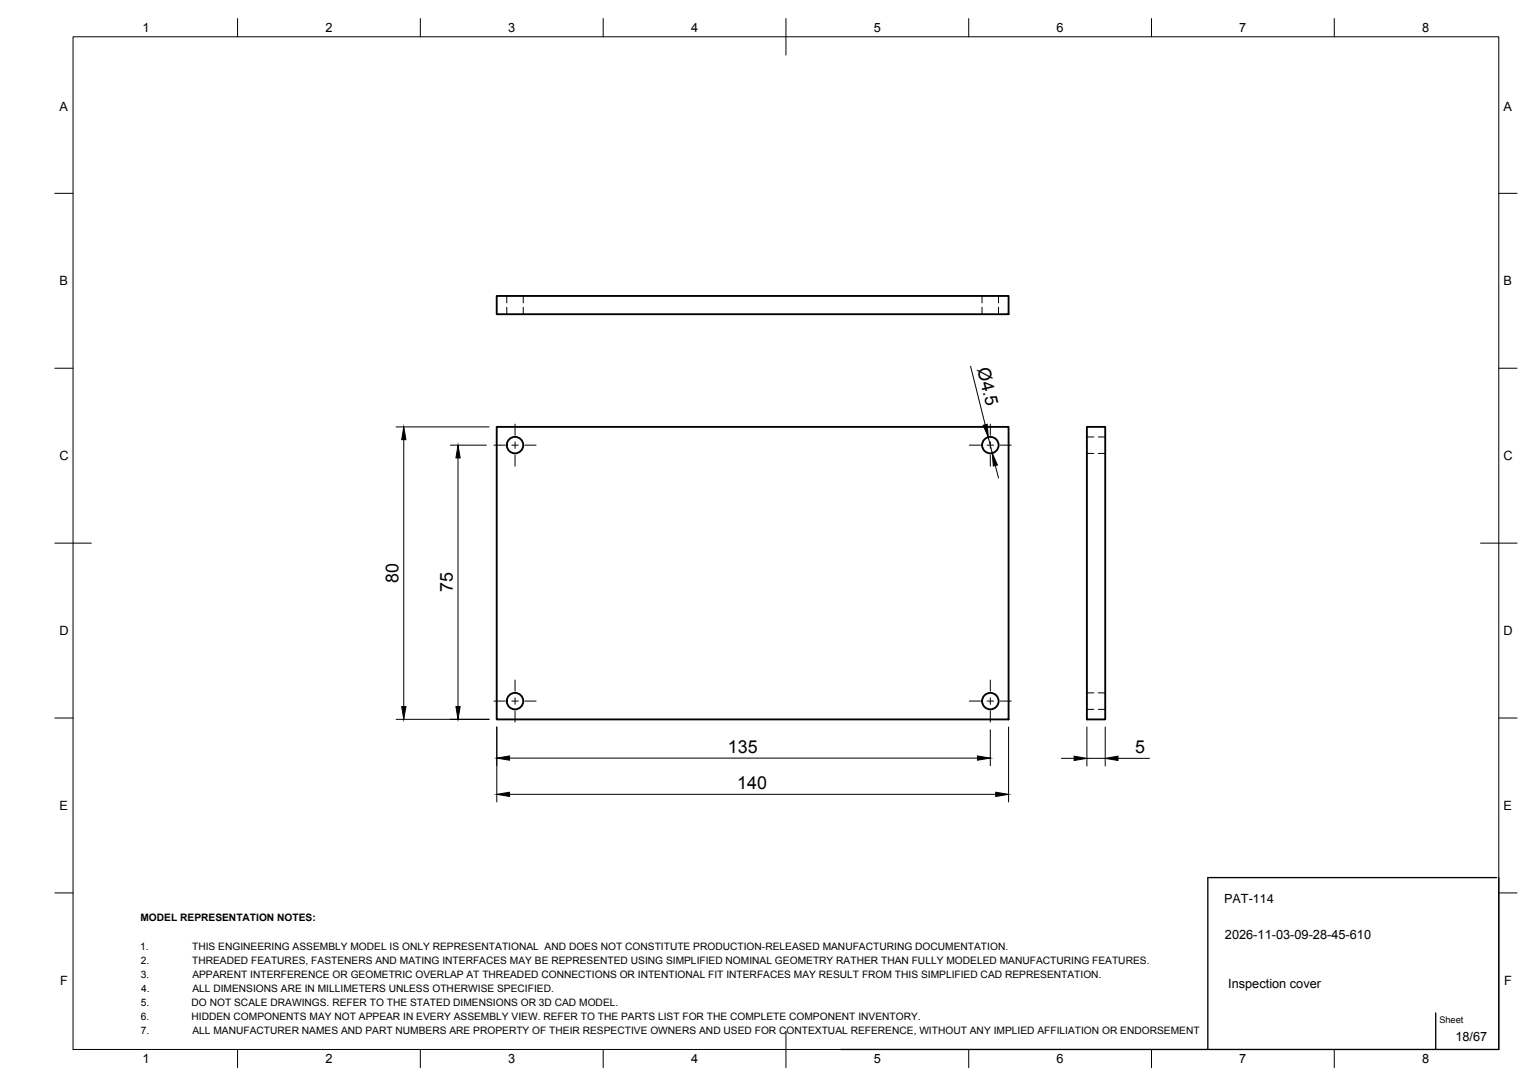
ISO-10303-21;
HEADER;
/* Generated by software containing ST-Developer
 * from STEP Tools, Inc. (www.steptools.com) 
 */

FILE_DESCRIPTION(
/* description */ ('Two-stage gear reducer in split housing'),
/* implementation_level */ '2;1');

FILE_NAME(
/* name */ 'Inspection cover.step',
/* time_stamp */ '2026-10-28T03:22:31-07:00',
/* author */ (''),
/* organization */ (''),
/* preprocessor_version */ 'ST-DEVELOPER v20.2',
/* originating_system */ 'Autodesk Translation Framework v15.17.0.0',
/* authorisation */ '');

FILE_SCHEMA (('AUTOMOTIVE_DESIGN { 1 0 10303 214 3 1 1 }'));
ENDSEC;

DATA;
#10=MECHANICAL_DESIGN_GEOMETRIC_PRESENTATION_REPRESENTATION('',(#1247),#73366);
#1135=SHAPE_REPRESENTATION_RELATIONSHIP('SRR','None',#73622,#1191);
#1191=ADVANCED_BREP_SHAPE_REPRESENTATION('',(#1318),#73318);
#1247=STYLED_ITEM('',(#73974),#1318);
#1318=MANIFOLD_SOLID_BREP('Body1',#16135);
#1510=FACE_BOUND('',#3320,.T.);
#1511=FACE_BOUND('',#3321,.T.);
#1512=FACE_BOUND('',#3322,.T.);
#1513=FACE_BOUND('',#3323,.T.);
#1514=FACE_BOUND('',#3325,.T.);
#1515=FACE_BOUND('',#3326,.T.);
#1516=FACE_BOUND('',#3327,.T.);
#1517=FACE_BOUND('',#3328,.T.);
#1726=PLANE('',#17372);
#1727=PLANE('',#17373);
#1728=PLANE('',#17374);
#1729=PLANE('',#17375);
#1730=PLANE('',#17376);
#1731=PLANE('',#17377);
#2262=FACE_OUTER_BOUND('',#3311,.T.);
#2263=FACE_OUTER_BOUND('',#3312,.T.);
#2264=FACE_OUTER_BOUND('',#3313,.T.);
#2265=FACE_OUTER_BOUND('',#3314,.T.);
#2266=FACE_OUTER_BOUND('',#3315,.T.);
#2267=FACE_OUTER_BOUND('',#3316,.T.);
#2268=FACE_OUTER_BOUND('',#3317,.T.);
#2269=FACE_OUTER_BOUND('',#3318,.T.);
#2270=FACE_OUTER_BOUND('',#3319,.T.);
#2271=FACE_OUTER_BOUND('',#3324,.T.);
#3311=EDGE_LOOP('',(#11659,#11660,#11661,#11662));
#3312=EDGE_LOOP('',(#11663,#11664,#11665,#11666));
#3313=EDGE_LOOP('',(#11667,#11668,#11669,#11670));
#3314=EDGE_LOOP('',(#11671,#11672,#11673,#11674));
#3315=EDGE_LOOP('',(#11675,#11676,#11677,#11678));
#3316=EDGE_LOOP('',(#11679,#11680,#11681,#11682));
#3317=EDGE_LOOP('',(#11683,#11684,#11685,#11686));
#3318=EDGE_LOOP('',(#11687,#11688,#11689,#11690));
#3319=EDGE_LOOP('',(#11691,#11692,#11693,#11694));
#3320=EDGE_LOOP('',(#11695));
#3321=EDGE_LOOP('',(#11696));
#3322=EDGE_LOOP('',(#11697));
#3323=EDGE_LOOP('',(#11698));
#3324=EDGE_LOOP('',(#11699,#11700,#11701,#11702));
#3325=EDGE_LOOP('',(#11703));
#3326=EDGE_LOOP('',(#11704));
#3327=EDGE_LOOP('',(#11705));
#3328=EDGE_LOOP('',(#11706));
#4360=LINE('',#24014,#5384);
#4361=LINE('',#24020,#5385);
#4362=LINE('',#24026,#5386);
#4363=LINE('',#24032,#5387);
#4364=LINE('',#24037,#5388);
#4365=LINE('',#24039,#5389);
#4366=LINE('',#24041,#5390);
#4367=LINE('',#24042,#5391);
#4368=LINE('',#24045,#5392);
#4369=LINE('',#24047,#5393);
#4370=LINE('',#24048,#5394);
#4371=LINE('',#24051,#5395);
#4372=LINE('',#24053,#5396);
#4373=LINE('',#24054,#5397);
#4374=LINE('',#24056,#5398);
#4375=LINE('',#24057,#5399);
#5384=VECTOR('',#19862,0.225);
#5385=VECTOR('',#19869,0.225);
#5386=VECTOR('',#19876,0.225);
#5387=VECTOR('',#19883,0.225);
#5388=VECTOR('',#19888,1.);
#5389=VECTOR('',#19889,1.);
#5390=VECTOR('',#19890,1.);
#5391=VECTOR('',#19891,1.);
#5392=VECTOR('',#19894,1.);
#5393=VECTOR('',#19895,1.);
#5394=VECTOR('',#19896,1.);
#5395=VECTOR('',#19899,1.);
#5396=VECTOR('',#19900,1.);
#5397=VECTOR('',#19901,1.);
#5398=VECTOR('',#19904,1.);
#5399=VECTOR('',#19905,1.);
#6376=CIRCLE('',#17361,0.225);
#6377=CIRCLE('',#17362,0.225);
#6378=CIRCLE('',#17364,0.225);
#6379=CIRCLE('',#17365,0.225);
#6380=CIRCLE('',#17367,0.225);
#6381=CIRCLE('',#17368,0.225);
#6382=CIRCLE('',#17370,0.225);
#6383=CIRCLE('',#17371,0.225);
#7208=VERTEX_POINT('',#24011);
#7209=VERTEX_POINT('',#24013);
#7210=VERTEX_POINT('',#24017);
#7211=VERTEX_POINT('',#24019);
#7212=VERTEX_POINT('',#24023);
#7213=VERTEX_POINT('',#24025);
#7214=VERTEX_POINT('',#24029);
#7215=VERTEX_POINT('',#24031);
#7216=VERTEX_POINT('',#24035);
#7217=VERTEX_POINT('',#24036);
#7218=VERTEX_POINT('',#24038);
#7219=VERTEX_POINT('',#24040);
#7220=VERTEX_POINT('',#24044);
#7221=VERTEX_POINT('',#24046);
#7222=VERTEX_POINT('',#24050);
#7223=VERTEX_POINT('',#24052);
#8883=EDGE_CURVE('',#7208,#7208,#6376,.T.);
#8884=EDGE_CURVE('',#7208,#7209,#4360,.T.);
#8885=EDGE_CURVE('',#7209,#7209,#6377,.T.);
#8886=EDGE_CURVE('',#7210,#7210,#6378,.T.);
#8887=EDGE_CURVE('',#7210,#7211,#4361,.T.);
#8888=EDGE_CURVE('',#7211,#7211,#6379,.T.);
#8889=EDGE_CURVE('',#7212,#7212,#6380,.T.);
#8890=EDGE_CURVE('',#7212,#7213,#4362,.T.);
#8891=EDGE_CURVE('',#7213,#7213,#6381,.T.);
#8892=EDGE_CURVE('',#7214,#7214,#6382,.T.);
#8893=EDGE_CURVE('',#7214,#7215,#4363,.T.);
#8894=EDGE_CURVE('',#7215,#7215,#6383,.T.);
#8895=EDGE_CURVE('',#7216,#7217,#4364,.T.);
#8896=EDGE_CURVE('',#7217,#7218,#4365,.T.);
#8897=EDGE_CURVE('',#7219,#7218,#4366,.T.);
#8898=EDGE_CURVE('',#7216,#7219,#4367,.T.);
#8899=EDGE_CURVE('',#7220,#7216,#4368,.T.);
#8900=EDGE_CURVE('',#7221,#7219,#4369,.T.);
#8901=EDGE_CURVE('',#7220,#7221,#4370,.T.);
#8902=EDGE_CURVE('',#7222,#7220,#4371,.T.);
#8903=EDGE_CURVE('',#7223,#7221,#4372,.T.);
#8904=EDGE_CURVE('',#7222,#7223,#4373,.T.);
#8905=EDGE_CURVE('',#7217,#7222,#4374,.T.);
#8906=EDGE_CURVE('',#7218,#7223,#4375,.T.);
#11659=ORIENTED_EDGE('',*,*,#8883,.F.);
#11660=ORIENTED_EDGE('',*,*,#8884,.T.);
#11661=ORIENTED_EDGE('',*,*,#8885,.F.);
#11662=ORIENTED_EDGE('',*,*,#8884,.F.);
#11663=ORIENTED_EDGE('',*,*,#8886,.F.);
#11664=ORIENTED_EDGE('',*,*,#8887,.T.);
#11665=ORIENTED_EDGE('',*,*,#8888,.F.);
#11666=ORIENTED_EDGE('',*,*,#8887,.F.);
#11667=ORIENTED_EDGE('',*,*,#8889,.F.);
#11668=ORIENTED_EDGE('',*,*,#8890,.T.);
#11669=ORIENTED_EDGE('',*,*,#8891,.F.);
#11670=ORIENTED_EDGE('',*,*,#8890,.F.);
#11671=ORIENTED_EDGE('',*,*,#8892,.F.);
#11672=ORIENTED_EDGE('',*,*,#8893,.T.);
#11673=ORIENTED_EDGE('',*,*,#8894,.F.);
#11674=ORIENTED_EDGE('',*,*,#8893,.F.);
#11675=ORIENTED_EDGE('',*,*,#8895,.T.);
#11676=ORIENTED_EDGE('',*,*,#8896,.T.);
#11677=ORIENTED_EDGE('',*,*,#8897,.F.);
#11678=ORIENTED_EDGE('',*,*,#8898,.F.);
#11679=ORIENTED_EDGE('',*,*,#8899,.T.);
#11680=ORIENTED_EDGE('',*,*,#8898,.T.);
#11681=ORIENTED_EDGE('',*,*,#8900,.F.);
#11682=ORIENTED_EDGE('',*,*,#8901,.F.);
#11683=ORIENTED_EDGE('',*,*,#8902,.T.);
#11684=ORIENTED_EDGE('',*,*,#8901,.T.);
#11685=ORIENTED_EDGE('',*,*,#8903,.F.);
#11686=ORIENTED_EDGE('',*,*,#8904,.F.);
#11687=ORIENTED_EDGE('',*,*,#8905,.T.);
#11688=ORIENTED_EDGE('',*,*,#8904,.T.);
#11689=ORIENTED_EDGE('',*,*,#8906,.F.);
#11690=ORIENTED_EDGE('',*,*,#8896,.F.);
#11691=ORIENTED_EDGE('',*,*,#8906,.T.);
#11692=ORIENTED_EDGE('',*,*,#8903,.T.);
#11693=ORIENTED_EDGE('',*,*,#8900,.T.);
#11694=ORIENTED_EDGE('',*,*,#8897,.T.);
#11695=ORIENTED_EDGE('',*,*,#8885,.T.);
#11696=ORIENTED_EDGE('',*,*,#8888,.T.);
#11697=ORIENTED_EDGE('',*,*,#8891,.T.);
#11698=ORIENTED_EDGE('',*,*,#8894,.T.);
#11699=ORIENTED_EDGE('',*,*,#8905,.F.);
#11700=ORIENTED_EDGE('',*,*,#8895,.F.);
#11701=ORIENTED_EDGE('',*,*,#8899,.F.);
#11702=ORIENTED_EDGE('',*,*,#8902,.F.);
#11703=ORIENTED_EDGE('',*,*,#8883,.T.);
#11704=ORIENTED_EDGE('',*,*,#8886,.T.);
#11705=ORIENTED_EDGE('',*,*,#8889,.T.);
#11706=ORIENTED_EDGE('',*,*,#8892,.T.);
#15043=CYLINDRICAL_SURFACE('',#17360,0.225);
#15044=CYLINDRICAL_SURFACE('',#17363,0.225);
#15045=CYLINDRICAL_SURFACE('',#17366,0.225);
#15046=CYLINDRICAL_SURFACE('',#17369,0.225);
#15469=ADVANCED_FACE('',(#2262),#15043,.F.);
#15470=ADVANCED_FACE('',(#2263),#15044,.F.);
#15471=ADVANCED_FACE('',(#2264),#15045,.F.);
#15472=ADVANCED_FACE('',(#2265),#15046,.F.);
#15473=ADVANCED_FACE('',(#2266),#1726,.T.);
#15474=ADVANCED_FACE('',(#2267),#1727,.T.);
#15475=ADVANCED_FACE('',(#2268),#1728,.T.);
#15476=ADVANCED_FACE('',(#2269),#1729,.T.);
#15477=ADVANCED_FACE('',(#2270,#1510,#1511,#1512,#1513),#1730,.T.);
#15478=ADVANCED_FACE('',(#2271,#1514,#1515,#1516,#1517),#1731,.F.);
#16135=CLOSED_SHELL('',(#15469,#15470,#15471,#15472,#15473,#15474,#15475,
#15476,#15477,#15478));
#17359=AXIS2_PLACEMENT_3D('',#24009,#19856,#19857);
#17360=AXIS2_PLACEMENT_3D('',#24010,#19858,#19859);
#17361=AXIS2_PLACEMENT_3D('',#24012,#19860,#19861);
#17362=AXIS2_PLACEMENT_3D('',#24015,#19863,#19864);
#17363=AXIS2_PLACEMENT_3D('',#24016,#19865,#19866);
#17364=AXIS2_PLACEMENT_3D('',#24018,#19867,#19868);
#17365=AXIS2_PLACEMENT_3D('',#24021,#19870,#19871);
#17366=AXIS2_PLACEMENT_3D('',#24022,#19872,#19873);
#17367=AXIS2_PLACEMENT_3D('',#24024,#19874,#19875);
#17368=AXIS2_PLACEMENT_3D('',#24027,#19877,#19878);
#17369=AXIS2_PLACEMENT_3D('',#24028,#19879,#19880);
#17370=AXIS2_PLACEMENT_3D('',#24030,#19881,#19882);
#17371=AXIS2_PLACEMENT_3D('',#24033,#19884,#19885);
#17372=AXIS2_PLACEMENT_3D('',#24034,#19886,#19887);
#17373=AXIS2_PLACEMENT_3D('',#24043,#19892,#19893);
#17374=AXIS2_PLACEMENT_3D('',#24049,#19897,#19898);
#17375=AXIS2_PLACEMENT_3D('',#24055,#19902,#19903);
#17376=AXIS2_PLACEMENT_3D('',#24058,#19906,#19907);
#17377=AXIS2_PLACEMENT_3D('',#24059,#19908,#19909);
#19856=DIRECTION('axis',(0.,0.,1.));
#19857=DIRECTION('refdir',(1.,0.,0.));
#19858=DIRECTION('center_axis',(0.,0.,1.));
#19859=DIRECTION('ref_axis',(1.,0.,0.));
#19860=DIRECTION('center_axis',(0.,0.,1.));
#19861=DIRECTION('ref_axis',(1.,0.,0.));
#19862=DIRECTION('',(0.,0.,1.));
#19863=DIRECTION('center_axis',(0.,0.,-1.));
#19864=DIRECTION('ref_axis',(1.,0.,0.));
#19865=DIRECTION('center_axis',(0.,0.,1.));
#19866=DIRECTION('ref_axis',(1.,0.,0.));
#19867=DIRECTION('center_axis',(0.,0.,1.));
#19868=DIRECTION('ref_axis',(1.,0.,0.));
#19869=DIRECTION('',(0.,0.,1.));
#19870=DIRECTION('center_axis',(0.,0.,-1.));
#19871=DIRECTION('ref_axis',(1.,0.,0.));
#19872=DIRECTION('center_axis',(0.,0.,1.));
#19873=DIRECTION('ref_axis',(1.,0.,0.));
#19874=DIRECTION('center_axis',(0.,0.,1.));
#19875=DIRECTION('ref_axis',(1.,0.,0.));
#19876=DIRECTION('',(0.,0.,1.));
#19877=DIRECTION('center_axis',(0.,0.,-1.));
#19878=DIRECTION('ref_axis',(1.,0.,0.));
#19879=DIRECTION('center_axis',(0.,0.,1.));
#19880=DIRECTION('ref_axis',(1.,0.,0.));
#19881=DIRECTION('center_axis',(0.,0.,1.));
#19882=DIRECTION('ref_axis',(1.,0.,0.));
#19883=DIRECTION('',(0.,0.,1.));
#19884=DIRECTION('center_axis',(0.,0.,-1.));
#19885=DIRECTION('ref_axis',(1.,0.,0.));
#19886=DIRECTION('center_axis',(0.,1.,0.));
#19887=DIRECTION('ref_axis',(-1.,0.,0.));
#19888=DIRECTION('',(-1.,0.,0.));
#19889=DIRECTION('',(0.,0.,1.));
#19890=DIRECTION('',(-1.,0.,0.));
#19891=DIRECTION('',(0.,0.,1.));
#19892=DIRECTION('center_axis',(1.,0.,0.));
#19893=DIRECTION('ref_axis',(0.,1.,0.));
#19894=DIRECTION('',(0.,1.,0.));
#19895=DIRECTION('',(0.,1.,0.));
#19896=DIRECTION('',(0.,0.,1.));
#19897=DIRECTION('center_axis',(0.,-1.,0.));
#19898=DIRECTION('ref_axis',(1.,0.,0.));
#19899=DIRECTION('',(1.,0.,0.));
#19900=DIRECTION('',(1.,0.,0.));
#19901=DIRECTION('',(0.,0.,1.));
#19902=DIRECTION('center_axis',(-1.,0.,0.));
#19903=DIRECTION('ref_axis',(0.,-1.,0.));
#19904=DIRECTION('',(0.,-1.,0.));
#19905=DIRECTION('',(0.,-1.,0.));
#19906=DIRECTION('center_axis',(0.,0.,1.));
#19907=DIRECTION('ref_axis',(1.,0.,0.));
#19908=DIRECTION('center_axis',(0.,0.,1.));
#19909=DIRECTION('ref_axis',(1.,0.,0.));
#24009=CARTESIAN_POINT('',(0.,0.,0.));
#24010=CARTESIAN_POINT('Origin',(14.5,-3.5,15.9));
#24011=CARTESIAN_POINT('',(14.275,-3.5,16.));
#24012=CARTESIAN_POINT('Origin',(14.5,-3.5,16.));
#24013=CARTESIAN_POINT('',(14.275,-3.5,16.5));
#24014=CARTESIAN_POINT('',(14.275,-3.5,15.9));
#24015=CARTESIAN_POINT('Origin',(14.5,-3.5,16.5));
#24016=CARTESIAN_POINT('Origin',(1.5,3.5,15.9));
#24017=CARTESIAN_POINT('',(1.275,3.5,16.));
#24018=CARTESIAN_POINT('Origin',(1.5,3.5,16.));
#24019=CARTESIAN_POINT('',(1.275,3.5,16.5));
#24020=CARTESIAN_POINT('',(1.275,3.5,15.9));
#24021=CARTESIAN_POINT('Origin',(1.5,3.5,16.5));
#24022=CARTESIAN_POINT('Origin',(1.5,-3.5,15.9));
#24023=CARTESIAN_POINT('',(1.275,-3.5,16.));
#24024=CARTESIAN_POINT('Origin',(1.5,-3.5,16.));
#24025=CARTESIAN_POINT('',(1.275,-3.5,16.5));
#24026=CARTESIAN_POINT('',(1.275,-3.5,15.9));
#24027=CARTESIAN_POINT('Origin',(1.5,-3.5,16.5));
#24028=CARTESIAN_POINT('Origin',(14.5,3.5,15.9));
#24029=CARTESIAN_POINT('',(14.275,3.5,16.));
#24030=CARTESIAN_POINT('Origin',(14.5,3.5,16.));
#24031=CARTESIAN_POINT('',(14.275,3.5,16.5));
#24032=CARTESIAN_POINT('',(14.275,3.5,15.9));
#24033=CARTESIAN_POINT('Origin',(14.5,3.5,16.5));
#24034=CARTESIAN_POINT('Origin',(15.,4.,16.));
#24035=CARTESIAN_POINT('',(15.,4.,16.));
#24036=CARTESIAN_POINT('',(1.,4.,16.));
#24037=CARTESIAN_POINT('',(15.,4.,16.));
#24038=CARTESIAN_POINT('',(1.,4.,16.5));
#24039=CARTESIAN_POINT('',(1.,4.,16.));
#24040=CARTESIAN_POINT('',(15.,4.,16.5));
#24041=CARTESIAN_POINT('',(15.,4.,16.5));
#24042=CARTESIAN_POINT('',(15.,4.,16.));
#24043=CARTESIAN_POINT('Origin',(15.,-4.,16.));
#24044=CARTESIAN_POINT('',(15.,-4.,16.));
#24045=CARTESIAN_POINT('',(15.,-4.,16.));
#24046=CARTESIAN_POINT('',(15.,-4.,16.5));
#24047=CARTESIAN_POINT('',(15.,-4.,16.5));
#24048=CARTESIAN_POINT('',(15.,-4.,16.));
#24049=CARTESIAN_POINT('Origin',(1.,-4.,16.));
#24050=CARTESIAN_POINT('',(1.,-4.,16.));
#24051=CARTESIAN_POINT('',(1.,-4.,16.));
#24052=CARTESIAN_POINT('',(1.,-4.,16.5));
#24053=CARTESIAN_POINT('',(1.,-4.,16.5));
#24054=CARTESIAN_POINT('',(1.,-4.,16.));
#24055=CARTESIAN_POINT('Origin',(1.,4.,16.));
#24056=CARTESIAN_POINT('',(1.,4.,16.));
#24057=CARTESIAN_POINT('',(1.,4.,16.5));
#24058=CARTESIAN_POINT('Origin',(8.,0.,16.5));
#24059=CARTESIAN_POINT('Origin',(8.,0.,16.));
#73254=UNCERTAINTY_MEASURE_WITH_UNIT(LENGTH_MEASURE(0.001),#73367,
'DISTANCE_ACCURACY_VALUE',
'Maximum model space distance between geometric entities at asserted c
onnectivities');
#73302=UNCERTAINTY_MEASURE_WITH_UNIT(LENGTH_MEASURE(0.001),#73367,
'DISTANCE_ACCURACY_VALUE',
'Maximum model space distance between geometric entities at asserted c
onnectivities');
#73318=(
GEOMETRIC_REPRESENTATION_CONTEXT(3)
GLOBAL_UNCERTAINTY_ASSIGNED_CONTEXT((#73254))
GLOBAL_UNIT_ASSIGNED_CONTEXT((#73367,#73369,#73370))
REPRESENTATION_CONTEXT('','3D')
);
#73366=(
GEOMETRIC_REPRESENTATION_CONTEXT(3)
GLOBAL_UNCERTAINTY_ASSIGNED_CONTEXT((#73302))
GLOBAL_UNIT_ASSIGNED_CONTEXT((#73367,#73369,#73370))
REPRESENTATION_CONTEXT('','3D')
);
#73367=(
LENGTH_UNIT()
NAMED_UNIT(*)
SI_UNIT(.CENTI.,.METRE.)
);
#73369=(
NAMED_UNIT(*)
PLANE_ANGLE_UNIT()
SI_UNIT($,.RADIAN.)
);
#73370=(
NAMED_UNIT(*)
SI_UNIT($,.STERADIAN.)
SOLID_ANGLE_UNIT()
);
#73386=SHAPE_DEFINITION_REPRESENTATION(#73449,#73622);
#73449=PRODUCT_DEFINITION_SHAPE('',$,#73686);
#73622=SHAPE_REPRESENTATION('',(#17359),#73318);
#73670=PRODUCT_DEFINITION_CONTEXT('part definition',#73861,'design');
#73686=PRODUCT_DEFINITION('Inspection cover','Inspection cover',#73749,
#73670);
#73749=PRODUCT_DEFINITION_FORMATION('',$,#73878);
#73861=APPLICATION_CONTEXT(
'Core Data for Automotive Mechanical Design Process');
#73862=PRODUCT_CONTEXT('part definition',#73861,'mechanical');
#73878=PRODUCT('Inspection cover','Inspection cover','Inspection cover',
(#73862));
#73968=COLOUR_RGB('Light Blue',0.38,0.62,0.78);
#73969=FILL_AREA_STYLE_COLOUR('',#73968);
#73970=FILL_AREA_STYLE('',(#73969));
#73971=SURFACE_STYLE_FILL_AREA(#73970);
#73972=SURFACE_SIDE_STYLE('',(#73971));
#73973=SURFACE_STYLE_USAGE(.BOTH.,#73972);
#73974=PRESENTATION_STYLE_ASSIGNMENT((#73973));
ENDSEC;
END-ISO-10303-21;
